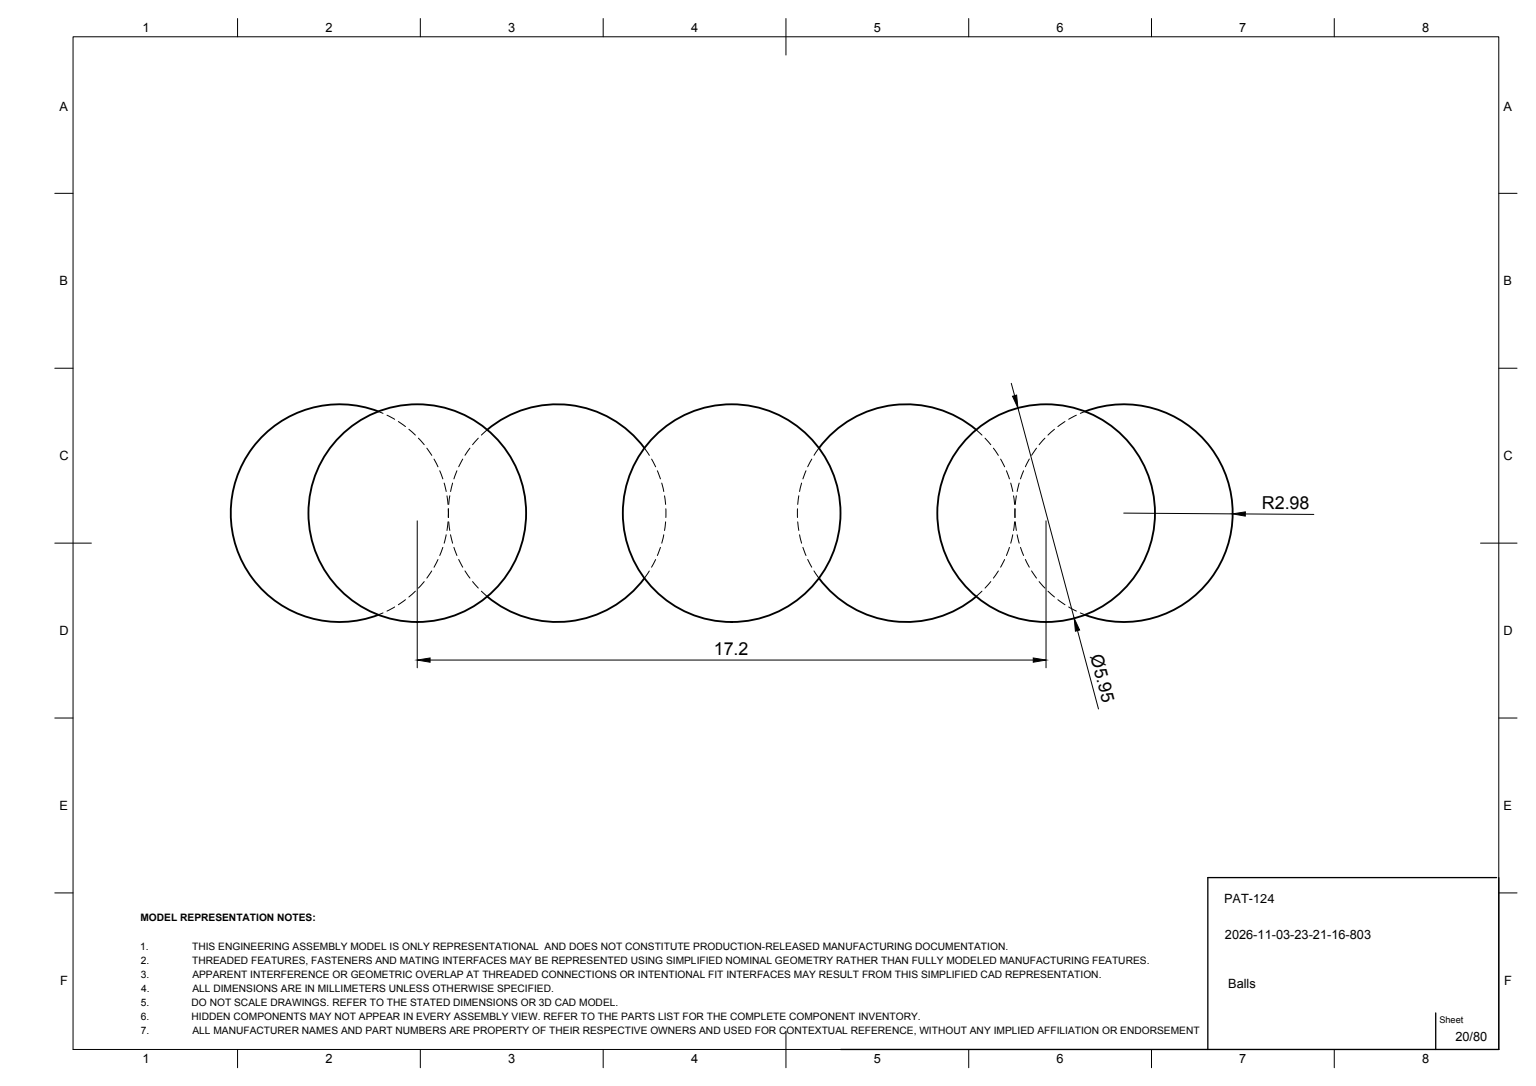
ISO-10303-21;
HEADER;
/* Generated by software containing ST-Developer
 * from STEP Tools, Inc. (www.steptools.com) 
 */

FILE_DESCRIPTION(
/* description */ ('XY cross-slide table'),
/* implementation_level */ '2;1');

FILE_NAME(
/* name */ 'Balls.step',
/* time_stamp */ '2026-10-28T03:22:46-07:00',
/* author */ (''),
/* organization */ (''),
/* preprocessor_version */ 'ST-DEVELOPER v20.2',
/* originating_system */ 'Autodesk Translation Framework v15.17.0.0',
/* authorisation */ '');

FILE_SCHEMA (('AUTOMOTIVE_DESIGN { 1 0 10303 214 3 1 1 }'));
ENDSEC;

DATA;
#10=MECHANICAL_DESIGN_GEOMETRIC_PRESENTATION_REPRESENTATION('',(#1683,#1684,#1685,#1686,#1687,#1688,#1689),#62984);
#1381=SPHERICAL_SURFACE('',#24327,0.29765);
#1382=SPHERICAL_SURFACE('',#24329,0.29765);
#1383=SPHERICAL_SURFACE('',#24331,0.29765);
#1384=SPHERICAL_SURFACE('',#24333,0.29765);
#1385=SPHERICAL_SURFACE('',#24335,0.29765);
#1386=SPHERICAL_SURFACE('',#24337,0.29765);
#1387=SPHERICAL_SURFACE('',#24339,0.29765);
#1517=SHAPE_REPRESENTATION_RELATIONSHIP('SRR','None',#63366,#1600);
#1600=ADVANCED_BREP_SHAPE_REPRESENTATION('',(#1796,#1797,#1798,#1799,#1800,
#1801,#1802),#62903);
#1683=STYLED_ITEM('',(#63912),#1796);
#1684=STYLED_ITEM('',(#63912),#1797);
#1685=STYLED_ITEM('',(#63912),#1798);
#1686=STYLED_ITEM('',(#63912),#1799);
#1687=STYLED_ITEM('',(#63912),#1800);
#1688=STYLED_ITEM('',(#63912),#1801);
#1689=STYLED_ITEM('',(#63912),#1802);
#1796=MANIFOLD_SOLID_BREP('Body1',#22977);
#1797=MANIFOLD_SOLID_BREP('Body2',#22978);
#1798=MANIFOLD_SOLID_BREP('Body3',#22979);
#1799=MANIFOLD_SOLID_BREP('Body4',#22980);
#1800=MANIFOLD_SOLID_BREP('Body5',#22981);
#1801=MANIFOLD_SOLID_BREP('Body6',#22982);
#1802=MANIFOLD_SOLID_BREP('Body7',#22983);
#3032=FACE_OUTER_BOUND('',#4446,.T.);
#3033=FACE_OUTER_BOUND('',#4447,.T.);
#3034=FACE_OUTER_BOUND('',#4448,.T.);
#3035=FACE_OUTER_BOUND('',#4449,.T.);
#3036=FACE_OUTER_BOUND('',#4450,.T.);
#3037=FACE_OUTER_BOUND('',#4451,.T.);
#3038=FACE_OUTER_BOUND('',#4452,.T.);
#4446=EDGE_LOOP('',(#15618,#15619));
#4447=EDGE_LOOP('',(#15620,#15621));
#4448=EDGE_LOOP('',(#15622,#15623));
#4449=EDGE_LOOP('',(#15624,#15625));
#4450=EDGE_LOOP('',(#15626,#15627));
#4451=EDGE_LOOP('',(#15628,#15629));
#4452=EDGE_LOOP('',(#15630,#15631));
#9026=CIRCLE('',#24328,0.29765);
#9027=CIRCLE('',#24330,0.29765);
#9028=CIRCLE('',#24332,0.29765);
#9029=CIRCLE('',#24334,0.29765);
#9030=CIRCLE('',#24336,0.29765);
#9031=CIRCLE('',#24338,0.29765);
#9032=CIRCLE('',#24340,0.29765);
#10007=VERTEX_POINT('',#33643);
#10008=VERTEX_POINT('',#33644);
#10009=VERTEX_POINT('',#33647);
#10010=VERTEX_POINT('',#33648);
#10011=VERTEX_POINT('',#33651);
#10012=VERTEX_POINT('',#33652);
#10013=VERTEX_POINT('',#33655);
#10014=VERTEX_POINT('',#33656);
#10015=VERTEX_POINT('',#33659);
#10016=VERTEX_POINT('',#33660);
#10017=VERTEX_POINT('',#33663);
#10018=VERTEX_POINT('',#33664);
#10019=VERTEX_POINT('',#33667);
#10020=VERTEX_POINT('',#33668);
#12193=EDGE_CURVE('',#10007,#10008,#9026,.T.);
#12194=EDGE_CURVE('',#10009,#10010,#9027,.T.);
#12195=EDGE_CURVE('',#10011,#10012,#9028,.T.);
#12196=EDGE_CURVE('',#10013,#10014,#9029,.T.);
#12197=EDGE_CURVE('',#10015,#10016,#9030,.T.);
#12198=EDGE_CURVE('',#10017,#10018,#9031,.T.);
#12199=EDGE_CURVE('',#10019,#10020,#9032,.T.);
#15618=ORIENTED_EDGE('',*,*,#12193,.T.);
#15619=ORIENTED_EDGE('',*,*,#12193,.F.);
#15620=ORIENTED_EDGE('',*,*,#12194,.T.);
#15621=ORIENTED_EDGE('',*,*,#12194,.F.);
#15622=ORIENTED_EDGE('',*,*,#12195,.T.);
#15623=ORIENTED_EDGE('',*,*,#12195,.F.);
#15624=ORIENTED_EDGE('',*,*,#12196,.T.);
#15625=ORIENTED_EDGE('',*,*,#12196,.F.);
#15626=ORIENTED_EDGE('',*,*,#12197,.T.);
#15627=ORIENTED_EDGE('',*,*,#12197,.F.);
#15628=ORIENTED_EDGE('',*,*,#12198,.T.);
#15629=ORIENTED_EDGE('',*,*,#12198,.F.);
#15630=ORIENTED_EDGE('',*,*,#12199,.T.);
#15631=ORIENTED_EDGE('',*,*,#12199,.F.);
#21813=ADVANCED_FACE('',(#3032),#1381,.T.);
#21814=ADVANCED_FACE('',(#3033),#1382,.T.);
#21815=ADVANCED_FACE('',(#3034),#1383,.T.);
#21816=ADVANCED_FACE('',(#3035),#1384,.T.);
#21817=ADVANCED_FACE('',(#3036),#1385,.T.);
#21818=ADVANCED_FACE('',(#3037),#1386,.T.);
#21819=ADVANCED_FACE('',(#3038),#1387,.T.);
#22977=CLOSED_SHELL('',(#21813));
#22978=CLOSED_SHELL('',(#21814));
#22979=CLOSED_SHELL('',(#21815));
#22980=CLOSED_SHELL('',(#21816));
#22981=CLOSED_SHELL('',(#21817));
#22982=CLOSED_SHELL('',(#21818));
#22983=CLOSED_SHELL('',(#21819));
#24326=AXIS2_PLACEMENT_3D('',#33641,#27324,#27325);
#24327=AXIS2_PLACEMENT_3D('',#33642,#27326,#27327);
#24328=AXIS2_PLACEMENT_3D('',#33645,#27328,#27329);
#24329=AXIS2_PLACEMENT_3D('',#33646,#27330,#27331);
#24330=AXIS2_PLACEMENT_3D('',#33649,#27332,#27333);
#24331=AXIS2_PLACEMENT_3D('',#33650,#27334,#27335);
#24332=AXIS2_PLACEMENT_3D('',#33653,#27336,#27337);
#24333=AXIS2_PLACEMENT_3D('',#33654,#27338,#27339);
#24334=AXIS2_PLACEMENT_3D('',#33657,#27340,#27341);
#24335=AXIS2_PLACEMENT_3D('',#33658,#27342,#27343);
#24336=AXIS2_PLACEMENT_3D('',#33661,#27344,#27345);
#24337=AXIS2_PLACEMENT_3D('',#33662,#27346,#27347);
#24338=AXIS2_PLACEMENT_3D('',#33665,#27348,#27349);
#24339=AXIS2_PLACEMENT_3D('',#33666,#27350,#27351);
#24340=AXIS2_PLACEMENT_3D('',#33669,#27352,#27353);
#27324=DIRECTION('axis',(0.,0.,1.));
#27325=DIRECTION('refdir',(1.,0.,0.));
#27326=DIRECTION('center_axis',(0.,0.,1.));
#27327=DIRECTION('ref_axis',(1.,0.,0.));
#27328=DIRECTION('center_axis',(1.22464679914735E-16,-1.,0.));
#27329=DIRECTION('ref_axis',(-1.,-1.22464679914735E-16,0.));
#27330=DIRECTION('center_axis',(0.78183148246803,0.,0.623489801858733));
#27331=DIRECTION('ref_axis',(0.623489801858734,0.,-0.78183148246803));
#27332=DIRECTION('center_axis',(7.63554790147315E-17,-1.,-9.57467422477103E-17));
#27333=DIRECTION('ref_axis',(-0.623489801858734,-1.22464679914735E-16,0.78183148246803));
#27334=DIRECTION('center_axis',(0.974927912181824,0.,-0.222520933956314));
#27335=DIRECTION('ref_axis',(-0.222520933956314,0.,-0.974927912181824));
#27336=DIRECTION('center_axis',(-2.7250954951288E-17,-1.,-1.19394234705288E-16));
#27337=DIRECTION('ref_axis',(0.222520933956314,-1.22464679914735E-16,0.974927912181824));
#27338=DIRECTION('center_axis',(0.433883739117558,0.,-0.900968867902419));
#27339=DIRECTION('ref_axis',(-0.900968867902419,0.,-0.433883739117558));
#27340=DIRECTION('center_axis',(-1.10336864020811E-16,-1.,-5.31354332312403E-17));
#27341=DIRECTION('ref_axis',(0.900968867902419,-1.22464679914735E-16,0.433883739117558));
#27342=DIRECTION('center_axis',(-0.433883739117558,0.,-0.900968867902419));
#27343=DIRECTION('ref_axis',(-0.900968867902419,0.,0.433883739117558));
#27344=DIRECTION('center_axis',(-1.10336864020811E-16,-1.,5.31354332312403E-17));
#27345=DIRECTION('ref_axis',(0.900968867902419,-1.22464679914735E-16,-0.433883739117558));
#27346=DIRECTION('center_axis',(-0.974927912181824,0.,-0.222520933956314));
#27347=DIRECTION('ref_axis',(-0.222520933956315,0.,0.974927912181824));
#27348=DIRECTION('center_axis',(-2.7250954951288E-17,-1.,1.19394234705288E-16));
#27349=DIRECTION('ref_axis',(0.222520933956315,-1.22464679914735E-16,-0.974927912181824));
#27350=DIRECTION('center_axis',(-0.78183148246803,0.,0.623489801858734));
#27351=DIRECTION('ref_axis',(0.623489801858733,0.,0.78183148246803));
#27352=DIRECTION('center_axis',(7.63554790147315E-17,-1.,9.57467422477103E-17));
#27353=DIRECTION('ref_axis',(-0.623489801858733,-1.22464679914735E-16,-0.78183148246803));
#33641=CARTESIAN_POINT('',(0.,0.,0.));
#33642=CARTESIAN_POINT('Origin',(1.1,0.,0.));
#33643=CARTESIAN_POINT('',(1.1,-2.23201749654651E-33,0.29765));
#33644=CARTESIAN_POINT('',(1.1,-2.23201749654651E-33,-0.29765));
#33645=CARTESIAN_POINT('Origin',(1.1,0.,0.));
#33646=CARTESIAN_POINT('Origin',(0.685838782044607,0.,-0.860014630714833));
#33647=CARTESIAN_POINT('',(0.918550922801216,-5.31350540756609E-33,-0.674432891191581));
#33648=CARTESIAN_POINT('',(0.453126641287998,8.49470414473068E-34,-1.04559637023808));
#33649=CARTESIAN_POINT('Origin',(0.685838782044607,0.,-0.860014630714833));
#33650=CARTESIAN_POINT('Origin',(-0.244773027351946,0.,-1.07242070340001));
#33651=CARTESIAN_POINT('',(0.0454142657089739,-2.23201749654651E-33,-1.1386540593921));
#33652=CARTESIAN_POINT('',(-0.534960320412865,-2.23201749654651E-33,-1.00618734740791));
#33653=CARTESIAN_POINT('Origin',(-0.244773027351946,0.,-1.07242070340001));
#33654=CARTESIAN_POINT('Origin',(-0.991065754692661,0.,-0.477272113029314));
#33655=CARTESIAN_POINT('',(-0.86192025974432,8.49470414473067E-34,-0.745445496560469));
#33656=CARTESIAN_POINT('',(-1.120211249641,-5.31350540756609E-33,-0.209098729498159));
#33657=CARTESIAN_POINT('Origin',(-0.991065754692661,0.,-0.477272113029314));
#33658=CARTESIAN_POINT('Origin',(-0.991065754692661,0.,0.477272113029314));
#33659=CARTESIAN_POINT('',(-1.120211249641,-2.23201749654651E-33,0.209098729498159));
#33660=CARTESIAN_POINT('',(-0.86192025974432,-2.23201749654651E-33,0.745445496560469));
#33661=CARTESIAN_POINT('Origin',(-0.991065754692661,0.,0.477272113029314));
#33662=CARTESIAN_POINT('Origin',(-0.244773027351946,0.,1.07242070340001));
#33663=CARTESIAN_POINT('',(-0.534960320412866,-2.23201749654651E-33,1.00618734740791));
#33664=CARTESIAN_POINT('',(0.0454142657089737,-2.23201749654651E-33,1.1386540593921));
#33665=CARTESIAN_POINT('Origin',(-0.244773027351946,0.,1.07242070340001));
#33666=CARTESIAN_POINT('Origin',(0.685838782044607,0.,0.860014630714833));
#33667=CARTESIAN_POINT('',(0.453126641287998,-2.23201749654651E-33,1.04559637023808));
#33668=CARTESIAN_POINT('',(0.918550922801216,-2.23201749654651E-33,0.674432891191581));
#33669=CARTESIAN_POINT('Origin',(0.685838782044607,0.,0.860014630714833));
#62804=UNCERTAINTY_MEASURE_WITH_UNIT(LENGTH_MEASURE(0.001),#62985,
'DISTANCE_ACCURACY_VALUE',
'Maximum model space distance between geometric entities at asserted c
onnectivities');
#62885=UNCERTAINTY_MEASURE_WITH_UNIT(LENGTH_MEASURE(0.001),#62985,
'DISTANCE_ACCURACY_VALUE',
'Maximum model space distance between geometric entities at asserted c
onnectivities');
#62903=(
GEOMETRIC_REPRESENTATION_CONTEXT(3)
GLOBAL_UNCERTAINTY_ASSIGNED_CONTEXT((#62804))
GLOBAL_UNIT_ASSIGNED_CONTEXT((#62985,#62987,#62988))
REPRESENTATION_CONTEXT('','3D')
);
#62984=(
GEOMETRIC_REPRESENTATION_CONTEXT(3)
GLOBAL_UNCERTAINTY_ASSIGNED_CONTEXT((#62885))
GLOBAL_UNIT_ASSIGNED_CONTEXT((#62985,#62987,#62988))
REPRESENTATION_CONTEXT('','3D')
);
#62985=(
LENGTH_UNIT()
NAMED_UNIT(*)
SI_UNIT(.CENTI.,.METRE.)
);
#62987=(
NAMED_UNIT(*)
PLANE_ANGLE_UNIT()
SI_UNIT($,.RADIAN.)
);
#62988=(
NAMED_UNIT(*)
SI_UNIT($,.STERADIAN.)
SOLID_ANGLE_UNIT()
);
#63006=SHAPE_DEFINITION_REPRESENTATION(#63104,#63366);
#63104=PRODUCT_DEFINITION_SHAPE('',$,#63465);
#63366=SHAPE_REPRESENTATION('',(#24326),#62903);
#63447=PRODUCT_DEFINITION_CONTEXT('part definition',#63743,'design');
#63465=PRODUCT_DEFINITION('Balls','Balls',#63563,#63447);
#63563=PRODUCT_DEFINITION_FORMATION('',$,#63762);
#63743=APPLICATION_CONTEXT(
'Core Data for Automotive Mechanical Design Process');
#63744=PRODUCT_CONTEXT('part definition',#63743,'mechanical');
#63762=PRODUCT('Balls','Balls','Balls',(#63744));
#63906=COLOUR_RGB('Grey',0.48,0.52,0.57);
#63907=FILL_AREA_STYLE_COLOUR('',#63906);
#63908=FILL_AREA_STYLE('',(#63907));
#63909=SURFACE_STYLE_FILL_AREA(#63908);
#63910=SURFACE_SIDE_STYLE('',(#63909));
#63911=SURFACE_STYLE_USAGE(.BOTH.,#63910);
#63912=PRESENTATION_STYLE_ASSIGNMENT((#63911));
ENDSEC;
END-ISO-10303-21;
